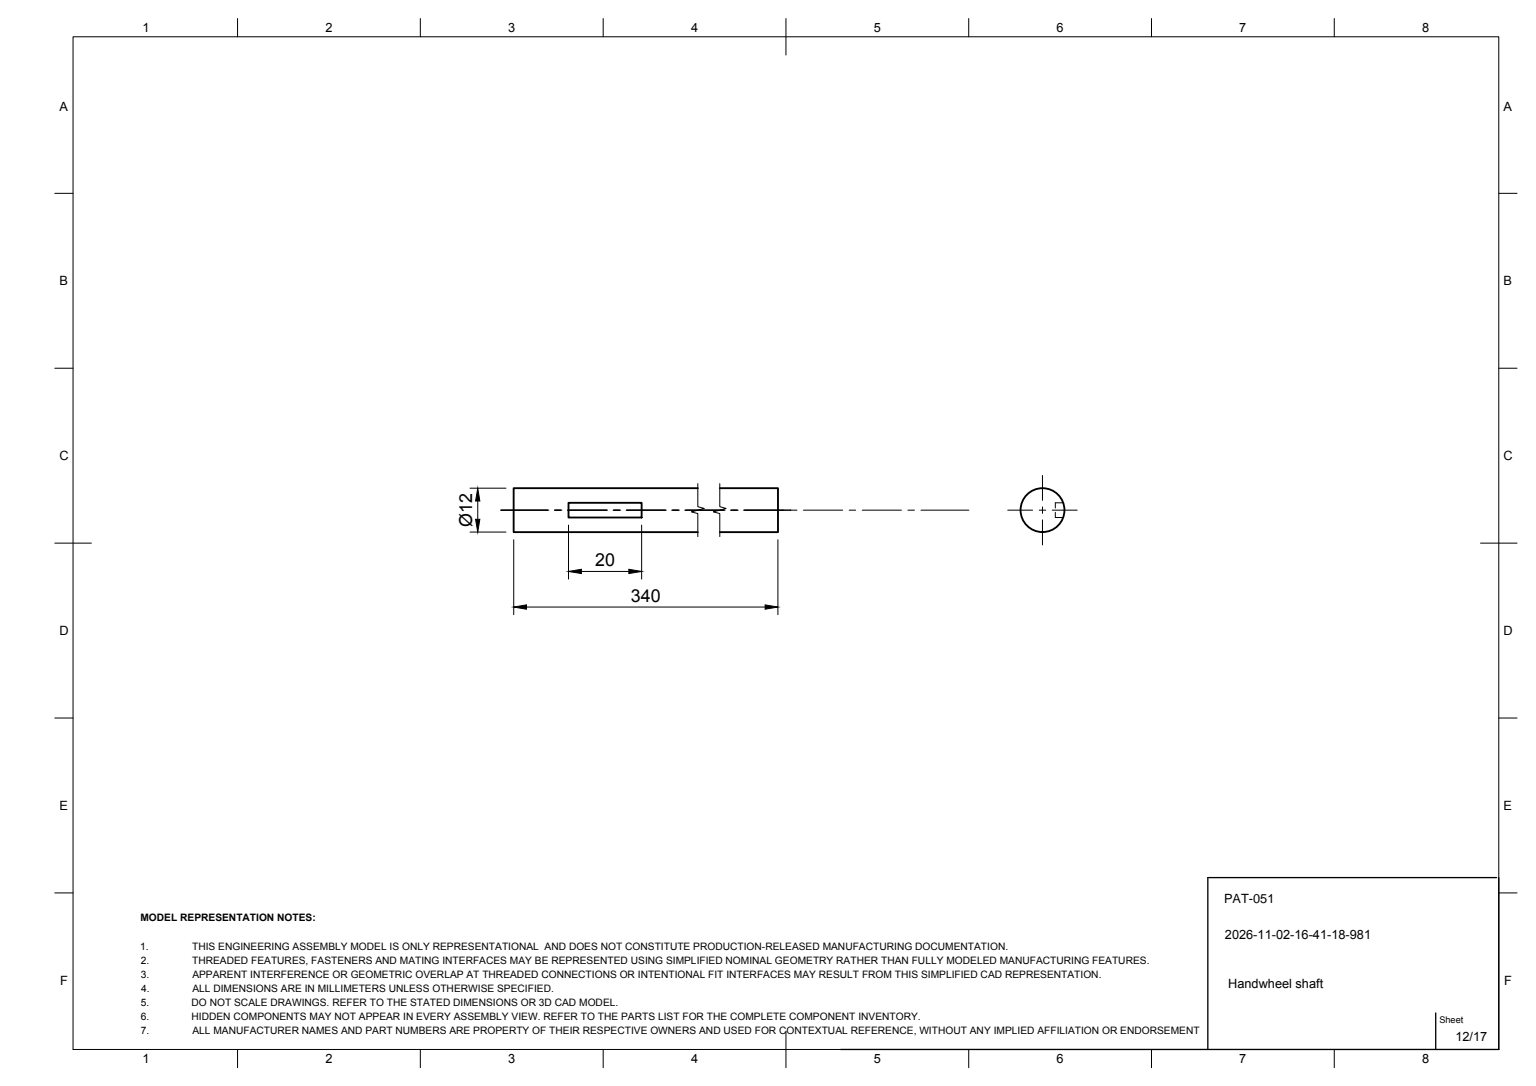
ISO-10303-21;
HEADER;
/* Generated by software containing ST-Developer
 * from STEP Tools, Inc. (www.steptools.com) 
 */

FILE_DESCRIPTION(
/* description */ ('Hand-crank flanged shaft unit'),
/* implementation_level */ '2;1');

FILE_NAME(
/* name */ 'Handwheel shaft.step',
/* time_stamp */ '2026-10-27T18:35:45-07:00',
/* author */ (''),
/* organization */ (''),
/* preprocessor_version */ 'ST-DEVELOPER v20.2',
/* originating_system */ 'Autodesk Translation Framework v15.17.0.0',
/* authorisation */ '');

FILE_SCHEMA (('AUTOMOTIVE_DESIGN { 1 0 10303 214 3 1 1 }'));
ENDSEC;

DATA;
#10=MECHANICAL_DESIGN_GEOMETRIC_PRESENTATION_REPRESENTATION('',(#293),#6805);
#252=SHAPE_REPRESENTATION_RELATIONSHIP('SRR','None',#6915,#272);
#272=ADVANCED_BREP_SHAPE_REPRESENTATION('',(#313),#6798);
#293=STYLED_ITEM('',(#7091),#313);
#313=MANIFOLD_SOLID_BREP('Body1',#3335);
#394=FACE_BOUND('',#899,.T.);
#472=PLANE('',#3807);
#473=PLANE('',#3808);
#474=PLANE('',#3810);
#475=PLANE('',#3811);
#476=PLANE('',#3812);
#477=PLANE('',#3817);
#478=PLANE('',#3818);
#631=FACE_OUTER_BOUND('',#893,.T.);
#632=FACE_OUTER_BOUND('',#894,.T.);
#633=FACE_OUTER_BOUND('',#895,.T.);
#634=FACE_OUTER_BOUND('',#896,.T.);
#635=FACE_OUTER_BOUND('',#897,.T.);
#636=FACE_OUTER_BOUND('',#898,.T.);
#637=FACE_OUTER_BOUND('',#900,.T.);
#638=FACE_OUTER_BOUND('',#901,.T.);
#893=EDGE_LOOP('',(#2743,#2744,#2745,#2746));
#894=EDGE_LOOP('',(#2747,#2748,#2749,#2750));
#895=EDGE_LOOP('',(#2751,#2752,#2753,#2754));
#896=EDGE_LOOP('',(#2755,#2756,#2757,#2758));
#897=EDGE_LOOP('',(#2759,#2760,#2761,#2762));
#898=EDGE_LOOP('',(#2763,#2764,#2765,#2766));
#899=EDGE_LOOP('',(#2767,#2768,#2769,#2770));
#900=EDGE_LOOP('',(#2771));
#901=EDGE_LOOP('',(#2772));
#1111=LINE('',#5922,#1339);
#1112=LINE('',#5924,#1340);
#1113=LINE('',#5926,#1341);
#1114=LINE('',#5927,#1342);
#1115=LINE('',#5932,#1343);
#1116=LINE('',#5933,#1344);
#1117=LINE('',#5936,#1345);
#1118=LINE('',#5937,#1346);
#1119=LINE('',#5940,#1347);
#1120=LINE('',#5941,#1348);
#1121=LINE('',#5948,#1349);
#1339=VECTOR('',#4578,1.);
#1340=VECTOR('',#4579,1.);
#1341=VECTOR('',#4580,1.);
#1342=VECTOR('',#4581,1.);
#1343=VECTOR('',#4586,1.);
#1344=VECTOR('',#4587,1.);
#1345=VECTOR('',#4590,1.);
#1346=VECTOR('',#4591,1.);
#1347=VECTOR('',#4594,1.);
#1348=VECTOR('',#4595,1.);
#1349=VECTOR('',#4604,0.6);
#1529=CIRCLE('',#3809,0.6);
#1530=CIRCLE('',#3813,0.6);
#1531=CIRCLE('',#3815,0.6);
#1532=CIRCLE('',#3816,0.6);
#1739=VERTEX_POINT('',#5920);
#1740=VERTEX_POINT('',#5921);
#1741=VERTEX_POINT('',#5923);
#1742=VERTEX_POINT('',#5925);
#1743=VERTEX_POINT('',#5929);
#1744=VERTEX_POINT('',#5931);
#1745=VERTEX_POINT('',#5935);
#1746=VERTEX_POINT('',#5939);
#1747=VERTEX_POINT('',#5945);
#1748=VERTEX_POINT('',#5947);
#2089=EDGE_CURVE('',#1739,#1740,#1111,.T.);
#2090=EDGE_CURVE('',#1739,#1741,#1112,.T.);
#2091=EDGE_CURVE('',#1741,#1742,#1113,.T.);
#2092=EDGE_CURVE('',#1742,#1740,#1114,.T.);
#2093=EDGE_CURVE('',#1740,#1743,#1529,.T.);
#2094=EDGE_CURVE('',#1744,#1742,#1115,.T.);
#2095=EDGE_CURVE('',#1743,#1744,#1116,.T.);
#2096=EDGE_CURVE('',#1741,#1745,#1117,.T.);
#2097=EDGE_CURVE('',#1745,#1744,#1118,.T.);
#2098=EDGE_CURVE('',#1743,#1746,#1119,.T.);
#2099=EDGE_CURVE('',#1745,#1746,#1120,.T.);
#2100=EDGE_CURVE('',#1746,#1739,#1530,.T.);
#2101=EDGE_CURVE('',#1747,#1747,#1531,.T.);
#2102=EDGE_CURVE('',#1747,#1748,#1121,.T.);
#2103=EDGE_CURVE('',#1748,#1748,#1532,.T.);
#2743=ORIENTED_EDGE('',*,*,#2089,.F.);
#2744=ORIENTED_EDGE('',*,*,#2090,.T.);
#2745=ORIENTED_EDGE('',*,*,#2091,.T.);
#2746=ORIENTED_EDGE('',*,*,#2092,.T.);
#2747=ORIENTED_EDGE('',*,*,#2093,.F.);
#2748=ORIENTED_EDGE('',*,*,#2092,.F.);
#2749=ORIENTED_EDGE('',*,*,#2094,.F.);
#2750=ORIENTED_EDGE('',*,*,#2095,.F.);
#2751=ORIENTED_EDGE('',*,*,#2096,.T.);
#2752=ORIENTED_EDGE('',*,*,#2097,.T.);
#2753=ORIENTED_EDGE('',*,*,#2094,.T.);
#2754=ORIENTED_EDGE('',*,*,#2091,.F.);
#2755=ORIENTED_EDGE('',*,*,#2098,.F.);
#2756=ORIENTED_EDGE('',*,*,#2095,.T.);
#2757=ORIENTED_EDGE('',*,*,#2097,.F.);
#2758=ORIENTED_EDGE('',*,*,#2099,.T.);
#2759=ORIENTED_EDGE('',*,*,#2100,.F.);
#2760=ORIENTED_EDGE('',*,*,#2099,.F.);
#2761=ORIENTED_EDGE('',*,*,#2096,.F.);
#2762=ORIENTED_EDGE('',*,*,#2090,.F.);
#2763=ORIENTED_EDGE('',*,*,#2101,.F.);
#2764=ORIENTED_EDGE('',*,*,#2102,.T.);
#2765=ORIENTED_EDGE('',*,*,#2103,.T.);
#2766=ORIENTED_EDGE('',*,*,#2102,.F.);
#2767=ORIENTED_EDGE('',*,*,#2098,.T.);
#2768=ORIENTED_EDGE('',*,*,#2100,.T.);
#2769=ORIENTED_EDGE('',*,*,#2089,.T.);
#2770=ORIENTED_EDGE('',*,*,#2093,.T.);
#2771=ORIENTED_EDGE('',*,*,#2101,.T.);
#2772=ORIENTED_EDGE('',*,*,#2103,.F.);
#3115=CYLINDRICAL_SURFACE('',#3814,0.6);
#3248=ADVANCED_FACE('',(#631),#472,.F.);
#3249=ADVANCED_FACE('',(#632),#473,.F.);
#3250=ADVANCED_FACE('',(#633),#474,.F.);
#3251=ADVANCED_FACE('',(#634),#475,.F.);
#3252=ADVANCED_FACE('',(#635),#476,.T.);
#3253=ADVANCED_FACE('',(#636,#394),#3115,.T.);
#3254=ADVANCED_FACE('',(#637),#477,.T.);
#3255=ADVANCED_FACE('',(#638),#478,.F.);
#3335=CLOSED_SHELL('',(#3248,#3249,#3250,#3251,#3252,#3253,#3254,#3255));
#3806=AXIS2_PLACEMENT_3D('',#5918,#4574,#4575);
#3807=AXIS2_PLACEMENT_3D('',#5919,#4576,#4577);
#3808=AXIS2_PLACEMENT_3D('',#5928,#4582,#4583);
#3809=AXIS2_PLACEMENT_3D('',#5930,#4584,#4585);
#3810=AXIS2_PLACEMENT_3D('',#5934,#4588,#4589);
#3811=AXIS2_PLACEMENT_3D('',#5938,#4592,#4593);
#3812=AXIS2_PLACEMENT_3D('',#5942,#4596,#4597);
#3813=AXIS2_PLACEMENT_3D('',#5943,#4598,#4599);
#3814=AXIS2_PLACEMENT_3D('',#5944,#4600,#4601);
#3815=AXIS2_PLACEMENT_3D('',#5946,#4602,#4603);
#3816=AXIS2_PLACEMENT_3D('',#5949,#4605,#4606);
#3817=AXIS2_PLACEMENT_3D('',#5950,#4607,#4608);
#3818=AXIS2_PLACEMENT_3D('',#5951,#4609,#4610);
#4574=DIRECTION('axis',(0.,0.,1.));
#4575=DIRECTION('refdir',(1.,0.,0.));
#4576=DIRECTION('center_axis',(-1.,0.,0.));
#4577=DIRECTION('ref_axis',(0.,0.,1.));
#4578=DIRECTION('',(0.,1.,0.));
#4579=DIRECTION('',(0.,0.,-1.));
#4580=DIRECTION('',(0.,1.,0.));
#4581=DIRECTION('',(0.,0.,1.));
#4582=DIRECTION('center_axis',(0.,1.,0.));
#4583=DIRECTION('ref_axis',(0.,0.,1.));
#4584=DIRECTION('center_axis',(0.,1.,0.));
#4585=DIRECTION('ref_axis',(1.,0.,0.));
#4586=DIRECTION('',(-1.,0.,0.));
#4587=DIRECTION('',(0.,0.,-1.));
#4588=DIRECTION('center_axis',(0.,0.,-1.));
#4589=DIRECTION('ref_axis',(-1.,0.,0.));
#4590=DIRECTION('',(1.,0.,0.));
#4591=DIRECTION('',(0.,1.,0.));
#4592=DIRECTION('center_axis',(1.,0.,0.));
#4593=DIRECTION('ref_axis',(0.,0.,-1.));
#4594=DIRECTION('',(0.,-1.,0.));
#4595=DIRECTION('',(0.,0.,1.));
#4596=DIRECTION('center_axis',(0.,1.,0.));
#4597=DIRECTION('ref_axis',(1.,0.,0.));
#4598=DIRECTION('center_axis',(0.,-1.,0.));
#4599=DIRECTION('ref_axis',(1.,0.,0.));
#4600=DIRECTION('center_axis',(0.,1.,0.));
#4601=DIRECTION('ref_axis',(1.,0.,0.));
#4602=DIRECTION('center_axis',(0.,1.,0.));
#4603=DIRECTION('ref_axis',(1.,0.,0.));
#4604=DIRECTION('',(0.,-1.,0.));
#4605=DIRECTION('center_axis',(0.,1.,0.));
#4606=DIRECTION('ref_axis',(1.,0.,0.));
#4607=DIRECTION('center_axis',(0.,1.,0.));
#4608=DIRECTION('ref_axis',(1.,0.,0.));
#4609=DIRECTION('center_axis',(0.,1.,0.));
#4610=DIRECTION('ref_axis',(1.,0.,0.));
#5918=CARTESIAN_POINT('',(0.,0.,0.));
#5919=CARTESIAN_POINT('Origin',(-0.2,27.,7.85));
#5920=CARTESIAN_POINT('',(-0.2,27.,8.06568542494924));
#5921=CARTESIAN_POINT('',(-0.2,29.,8.06568542494924));
#5922=CARTESIAN_POINT('',(-0.2,-3.5,8.06568542494924));
#5923=CARTESIAN_POINT('',(-0.2,27.,7.85));
#5924=CARTESIAN_POINT('',(-0.2,27.,8.2));
#5925=CARTESIAN_POINT('',(-0.2,29.,7.85));
#5926=CARTESIAN_POINT('',(-0.2,27.,7.85));
#5927=CARTESIAN_POINT('',(-0.2,29.,8.2));
#5928=CARTESIAN_POINT('Origin',(0.,29.,8.025));
#5929=CARTESIAN_POINT('',(0.2,29.,8.06568542494924));
#5930=CARTESIAN_POINT('Origin',(0.,29.,7.5));
#5931=CARTESIAN_POINT('',(0.2,29.,7.85));
#5932=CARTESIAN_POINT('',(-0.2,29.,7.85));
#5933=CARTESIAN_POINT('',(0.2,29.,7.85));
#5934=CARTESIAN_POINT('Origin',(0.2,27.,7.85));
#5935=CARTESIAN_POINT('',(0.2,27.,7.85));
#5936=CARTESIAN_POINT('',(-0.2,27.,7.85));
#5937=CARTESIAN_POINT('',(0.2,27.,7.85));
#5938=CARTESIAN_POINT('Origin',(0.2,27.,8.2));
#5939=CARTESIAN_POINT('',(0.2,27.,8.06568542494924));
#5940=CARTESIAN_POINT('',(0.2,-3.5,8.06568542494924));
#5941=CARTESIAN_POINT('',(0.2,27.,7.85));
#5942=CARTESIAN_POINT('Origin',(0.,27.,8.025));
#5943=CARTESIAN_POINT('Origin',(0.,27.,7.5));
#5944=CARTESIAN_POINT('Origin',(0.,-3.5,7.5));
#5945=CARTESIAN_POINT('',(-0.6,30.5,7.5));
#5946=CARTESIAN_POINT('Origin',(0.,30.5,7.5));
#5947=CARTESIAN_POINT('',(-0.6,-3.5,7.5));
#5948=CARTESIAN_POINT('',(-0.6,-3.5,7.5));
#5949=CARTESIAN_POINT('Origin',(0.,-3.5,7.5));
#5950=CARTESIAN_POINT('Origin',(0.,30.5,7.5));
#5951=CARTESIAN_POINT('Origin',(0.,-3.5,7.5));
#6773=UNCERTAINTY_MEASURE_WITH_UNIT(LENGTH_MEASURE(0.001),#6806,
'DISTANCE_ACCURACY_VALUE',
'Maximum model space distance between geometric entities at asserted c
onnectivities');
#6780=UNCERTAINTY_MEASURE_WITH_UNIT(LENGTH_MEASURE(0.001),#6806,
'DISTANCE_ACCURACY_VALUE',
'Maximum model space distance between geometric entities at asserted c
onnectivities');
#6798=(
GEOMETRIC_REPRESENTATION_CONTEXT(3)
GLOBAL_UNCERTAINTY_ASSIGNED_CONTEXT((#6773))
GLOBAL_UNIT_ASSIGNED_CONTEXT((#6806,#6808,#6809))
REPRESENTATION_CONTEXT('','3D')
);
#6805=(
GEOMETRIC_REPRESENTATION_CONTEXT(3)
GLOBAL_UNCERTAINTY_ASSIGNED_CONTEXT((#6780))
GLOBAL_UNIT_ASSIGNED_CONTEXT((#6806,#6808,#6809))
REPRESENTATION_CONTEXT('','3D')
);
#6806=(
LENGTH_UNIT()
NAMED_UNIT(*)
SI_UNIT(.CENTI.,.METRE.)
);
#6808=(
NAMED_UNIT(*)
PLANE_ANGLE_UNIT()
SI_UNIT($,.RADIAN.)
);
#6809=(
NAMED_UNIT(*)
SI_UNIT($,.STERADIAN.)
SOLID_ANGLE_UNIT()
);
#6827=SHAPE_DEFINITION_REPRESENTATION(#6880,#6915);
#6880=PRODUCT_DEFINITION_SHAPE('',$,#6940);
#6915=SHAPE_REPRESENTATION('',(#3806),#6798);
#6922=PRODUCT_DEFINITION_CONTEXT('part definition',#6996,'design');
#6940=PRODUCT_DEFINITION('Handwheel shaft','Handwheel shaft',#6964,#6922);
#6964=PRODUCT_DEFINITION_FORMATION('',$,#7015);
#6996=APPLICATION_CONTEXT(
'Core Data for Automotive Mechanical Design Process');
#6997=PRODUCT_CONTEXT('part definition',#6996,'mechanical');
#7015=PRODUCT('Handwheel shaft','Handwheel shaft','Handwheel shaft',(#6997));
#7085=COLOUR_RGB('Grey',0.48,0.52,0.57);
#7086=FILL_AREA_STYLE_COLOUR('',#7085);
#7087=FILL_AREA_STYLE('',(#7086));
#7088=SURFACE_STYLE_FILL_AREA(#7087);
#7089=SURFACE_SIDE_STYLE('',(#7088));
#7090=SURFACE_STYLE_USAGE(.BOTH.,#7089);
#7091=PRESENTATION_STYLE_ASSIGNMENT((#7090));
ENDSEC;
END-ISO-10303-21;
